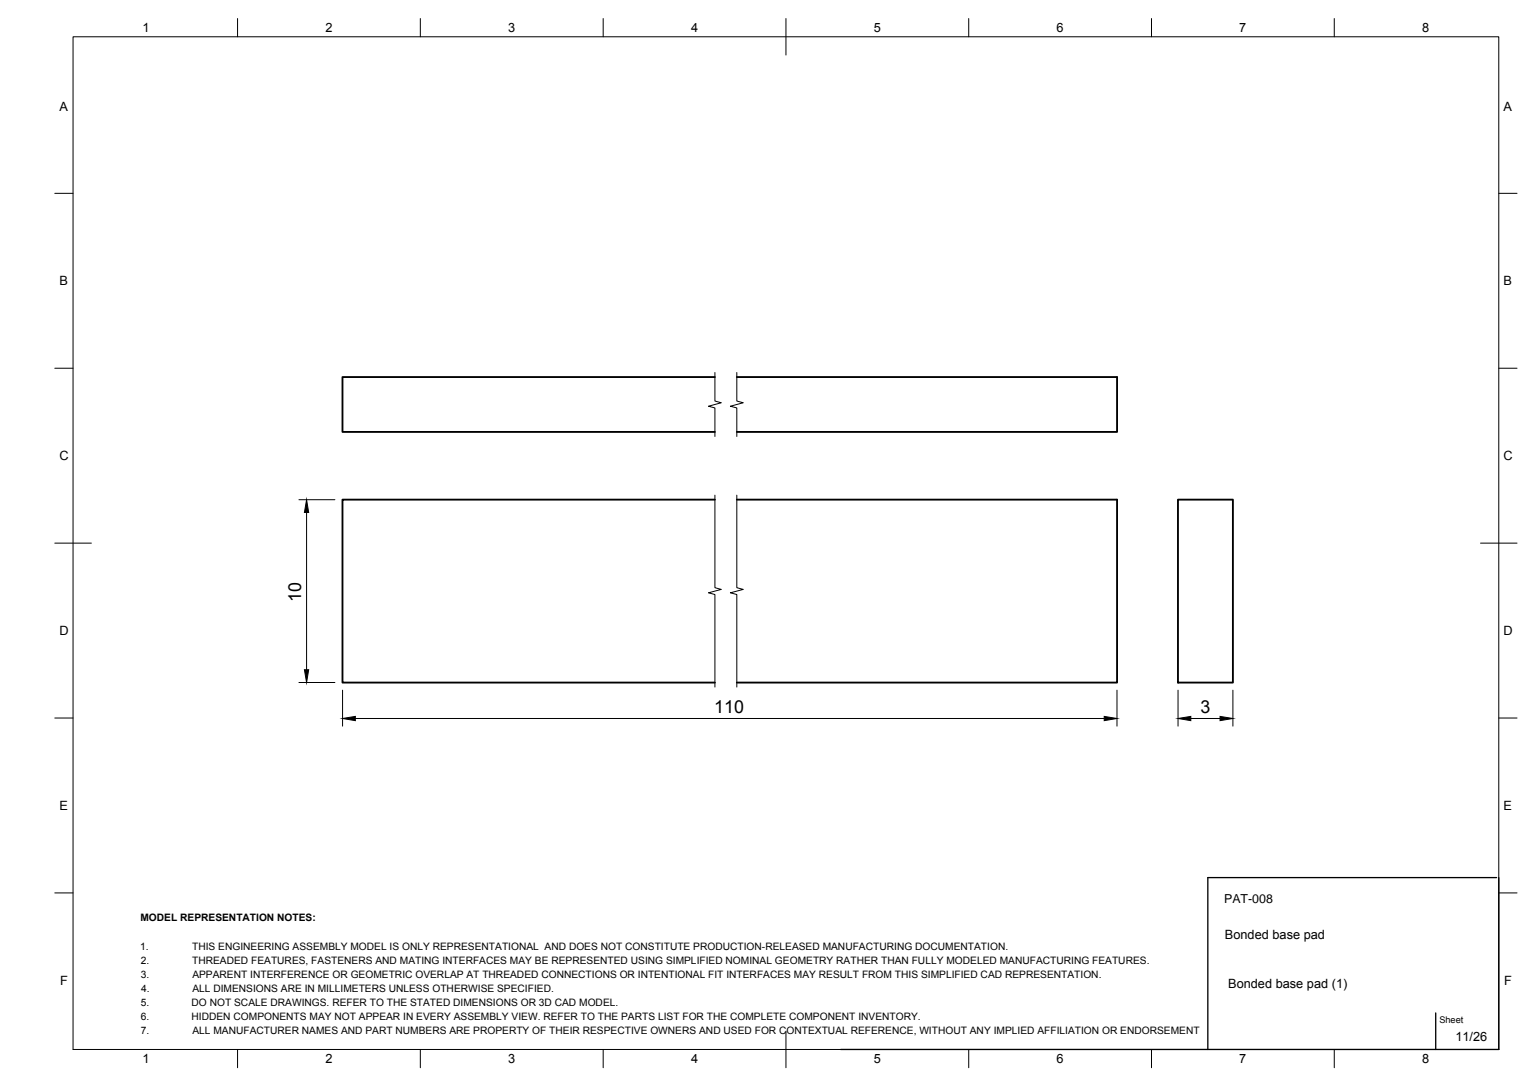
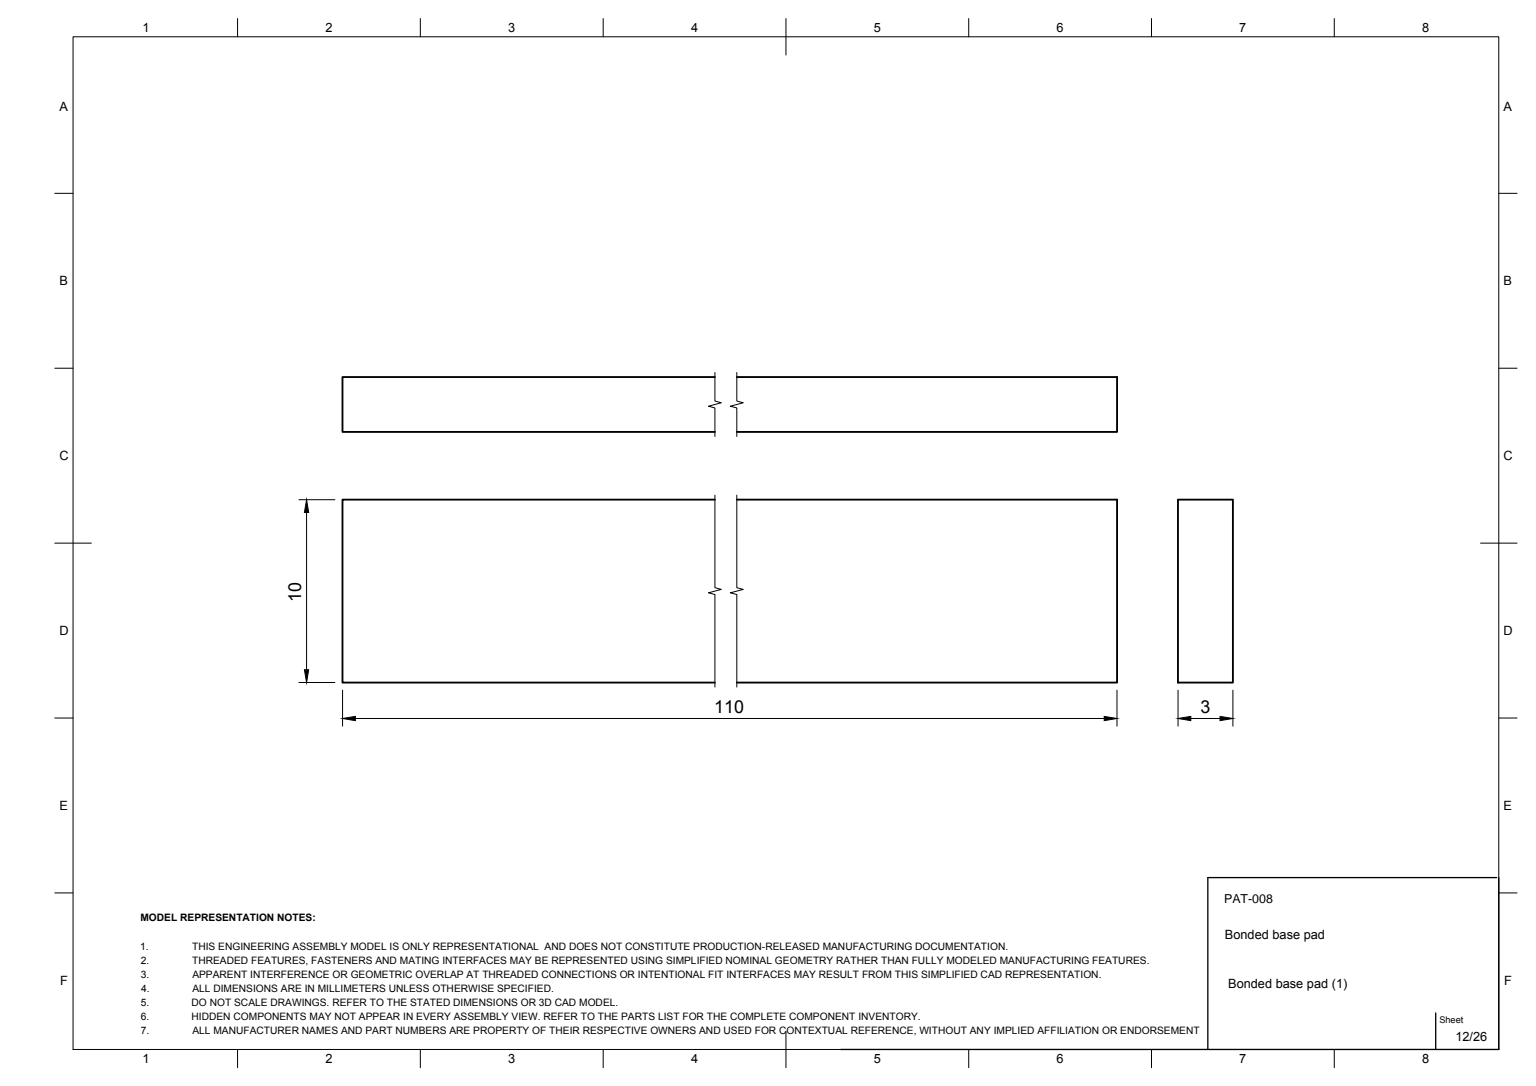
ISO-10303-21;
HEADER;
/* Generated by software containing ST-Developer
 * from STEP Tools, Inc. (www.steptools.com) 
 */

FILE_DESCRIPTION(
/* description */ ('Bearing housing with oil seal and end cap'),
/* implementation_level */ '2;1');

FILE_NAME(
/* name */ 'Bonded base pad (1).step',
/* time_stamp */ '2026-10-28T03:23:10-07:00',
/* author */ (''),
/* organization */ (''),
/* preprocessor_version */ 'ST-DEVELOPER v20.2',
/* originating_system */ 'Autodesk Translation Framework v15.17.0.0',
/* authorisation */ '');

FILE_SCHEMA (('AUTOMOTIVE_DESIGN { 1 0 10303 214 3 1 1 }'));
ENDSEC;

DATA;
#10=MECHANICAL_DESIGN_GEOMETRIC_PRESENTATION_REPRESENTATION('',(#266),#7871);
#224=SHAPE_REPRESENTATION_RELATIONSHIP('SRR','None',#7971,#245);
#245=ADVANCED_BREP_SHAPE_REPRESENTATION('',(#295),#7855);
#266=STYLED_ITEM('',(#8132),#295);
#295=MANIFOLD_SOLID_BREP('Body1',#4092);
#465=PLANE('',#4549);
#466=PLANE('',#4550);
#467=PLANE('',#4551);
#468=PLANE('',#4552);
#469=PLANE('',#4553);
#470=PLANE('',#4554);
#651=FACE_OUTER_BOUND('',#961,.T.);
#652=FACE_OUTER_BOUND('',#962,.T.);
#653=FACE_OUTER_BOUND('',#963,.T.);
#654=FACE_OUTER_BOUND('',#964,.T.);
#655=FACE_OUTER_BOUND('',#965,.T.);
#656=FACE_OUTER_BOUND('',#966,.T.);
#961=EDGE_LOOP('',(#3131,#3132,#3133,#3134));
#962=EDGE_LOOP('',(#3135,#3136,#3137,#3138));
#963=EDGE_LOOP('',(#3139,#3140,#3141,#3142));
#964=EDGE_LOOP('',(#3143,#3144,#3145,#3146));
#965=EDGE_LOOP('',(#3147,#3148,#3149,#3150));
#966=EDGE_LOOP('',(#3151,#3152,#3153,#3154));
#1249=LINE('',#6640,#1511);
#1250=LINE('',#6642,#1512);
#1251=LINE('',#6644,#1513);
#1252=LINE('',#6645,#1514);
#1253=LINE('',#6648,#1515);
#1254=LINE('',#6650,#1516);
#1255=LINE('',#6651,#1517);
#1256=LINE('',#6654,#1518);
#1257=LINE('',#6656,#1519);
#1258=LINE('',#6657,#1520);
#1259=LINE('',#6659,#1521);
#1260=LINE('',#6660,#1522);
#1511=VECTOR('',#5386,1.);
#1512=VECTOR('',#5387,1.);
#1513=VECTOR('',#5388,1.);
#1514=VECTOR('',#5389,1.);
#1515=VECTOR('',#5392,1.);
#1516=VECTOR('',#5393,1.);
#1517=VECTOR('',#5394,1.);
#1518=VECTOR('',#5397,1.);
#1519=VECTOR('',#5398,1.);
#1520=VECTOR('',#5399,1.);
#1521=VECTOR('',#5402,1.);
#1522=VECTOR('',#5403,1.);
#2019=VERTEX_POINT('',#6638);
#2020=VERTEX_POINT('',#6639);
#2021=VERTEX_POINT('',#6641);
#2022=VERTEX_POINT('',#6643);
#2023=VERTEX_POINT('',#6647);
#2024=VERTEX_POINT('',#6649);
#2025=VERTEX_POINT('',#6653);
#2026=VERTEX_POINT('',#6655);
#2429=EDGE_CURVE('',#2019,#2020,#1249,.T.);
#2430=EDGE_CURVE('',#2020,#2021,#1250,.T.);
#2431=EDGE_CURVE('',#2022,#2021,#1251,.T.);
#2432=EDGE_CURVE('',#2019,#2022,#1252,.T.);
#2433=EDGE_CURVE('',#2023,#2019,#1253,.T.);
#2434=EDGE_CURVE('',#2024,#2022,#1254,.T.);
#2435=EDGE_CURVE('',#2023,#2024,#1255,.T.);
#2436=EDGE_CURVE('',#2025,#2023,#1256,.T.);
#2437=EDGE_CURVE('',#2026,#2024,#1257,.T.);
#2438=EDGE_CURVE('',#2025,#2026,#1258,.T.);
#2439=EDGE_CURVE('',#2020,#2025,#1259,.T.);
#2440=EDGE_CURVE('',#2021,#2026,#1260,.T.);
#3131=ORIENTED_EDGE('',*,*,#2429,.T.);
#3132=ORIENTED_EDGE('',*,*,#2430,.T.);
#3133=ORIENTED_EDGE('',*,*,#2431,.F.);
#3134=ORIENTED_EDGE('',*,*,#2432,.F.);
#3135=ORIENTED_EDGE('',*,*,#2433,.T.);
#3136=ORIENTED_EDGE('',*,*,#2432,.T.);
#3137=ORIENTED_EDGE('',*,*,#2434,.F.);
#3138=ORIENTED_EDGE('',*,*,#2435,.F.);
#3139=ORIENTED_EDGE('',*,*,#2436,.T.);
#3140=ORIENTED_EDGE('',*,*,#2435,.T.);
#3141=ORIENTED_EDGE('',*,*,#2437,.F.);
#3142=ORIENTED_EDGE('',*,*,#2438,.F.);
#3143=ORIENTED_EDGE('',*,*,#2439,.T.);
#3144=ORIENTED_EDGE('',*,*,#2438,.T.);
#3145=ORIENTED_EDGE('',*,*,#2440,.F.);
#3146=ORIENTED_EDGE('',*,*,#2430,.F.);
#3147=ORIENTED_EDGE('',*,*,#2440,.T.);
#3148=ORIENTED_EDGE('',*,*,#2437,.T.);
#3149=ORIENTED_EDGE('',*,*,#2434,.T.);
#3150=ORIENTED_EDGE('',*,*,#2431,.T.);
#3151=ORIENTED_EDGE('',*,*,#2439,.F.);
#3152=ORIENTED_EDGE('',*,*,#2429,.F.);
#3153=ORIENTED_EDGE('',*,*,#2433,.F.);
#3154=ORIENTED_EDGE('',*,*,#2436,.F.);
#3933=ADVANCED_FACE('',(#651),#465,.T.);
#3934=ADVANCED_FACE('',(#652),#466,.T.);
#3935=ADVANCED_FACE('',(#653),#467,.T.);
#3936=ADVANCED_FACE('',(#654),#468,.T.);
#3937=ADVANCED_FACE('',(#655),#469,.T.);
#3938=ADVANCED_FACE('',(#656),#470,.F.);
#4092=CLOSED_SHELL('',(#3933,#3934,#3935,#3936,#3937,#3938));
#4548=AXIS2_PLACEMENT_3D('',#6636,#5382,#5383);
#4549=AXIS2_PLACEMENT_3D('',#6637,#5384,#5385);
#4550=AXIS2_PLACEMENT_3D('',#6646,#5390,#5391);
#4551=AXIS2_PLACEMENT_3D('',#6652,#5395,#5396);
#4552=AXIS2_PLACEMENT_3D('',#6658,#5400,#5401);
#4553=AXIS2_PLACEMENT_3D('',#6661,#5404,#5405);
#4554=AXIS2_PLACEMENT_3D('',#6662,#5406,#5407);
#5382=DIRECTION('axis',(0.,0.,1.));
#5383=DIRECTION('refdir',(1.,0.,0.));
#5384=DIRECTION('center_axis',(0.,1.,0.));
#5385=DIRECTION('ref_axis',(-1.,0.,0.));
#5386=DIRECTION('',(-1.,0.,0.));
#5387=DIRECTION('',(0.,0.,1.));
#5388=DIRECTION('',(-1.,0.,0.));
#5389=DIRECTION('',(0.,0.,1.));
#5390=DIRECTION('center_axis',(1.,0.,0.));
#5391=DIRECTION('ref_axis',(0.,1.,0.));
#5392=DIRECTION('',(0.,1.,0.));
#5393=DIRECTION('',(0.,1.,0.));
#5394=DIRECTION('',(0.,0.,1.));
#5395=DIRECTION('center_axis',(0.,-1.,0.));
#5396=DIRECTION('ref_axis',(1.,0.,0.));
#5397=DIRECTION('',(1.,0.,0.));
#5398=DIRECTION('',(1.,0.,0.));
#5399=DIRECTION('',(0.,0.,1.));
#5400=DIRECTION('center_axis',(-1.,0.,0.));
#5401=DIRECTION('ref_axis',(0.,-1.,0.));
#5402=DIRECTION('',(0.,-1.,0.));
#5403=DIRECTION('',(0.,-1.,0.));
#5404=DIRECTION('center_axis',(0.,0.,1.));
#5405=DIRECTION('ref_axis',(1.,0.,0.));
#5406=DIRECTION('center_axis',(0.,0.,1.));
#5407=DIRECTION('ref_axis',(1.,0.,0.));
#6636=CARTESIAN_POINT('',(0.,0.,0.));
#6637=CARTESIAN_POINT('Origin',(5.5,7.,-0.3));
#6638=CARTESIAN_POINT('',(5.5,7.,-0.3));
#6639=CARTESIAN_POINT('',(-5.5,7.,-0.3));
#6640=CARTESIAN_POINT('',(5.5,7.,-0.3));
#6641=CARTESIAN_POINT('',(-5.5,7.,0.));
#6642=CARTESIAN_POINT('',(-5.5,7.,-0.3));
#6643=CARTESIAN_POINT('',(5.5,7.,0.));
#6644=CARTESIAN_POINT('',(5.5,7.,0.));
#6645=CARTESIAN_POINT('',(5.5,7.,-0.3));
#6646=CARTESIAN_POINT('Origin',(5.5,6.,-0.3));
#6647=CARTESIAN_POINT('',(5.5,6.,-0.3));
#6648=CARTESIAN_POINT('',(5.5,6.,-0.3));
#6649=CARTESIAN_POINT('',(5.5,6.,0.));
#6650=CARTESIAN_POINT('',(5.5,6.,0.));
#6651=CARTESIAN_POINT('',(5.5,6.,-0.3));
#6652=CARTESIAN_POINT('Origin',(-5.5,6.,-0.3));
#6653=CARTESIAN_POINT('',(-5.5,6.,-0.3));
#6654=CARTESIAN_POINT('',(-5.5,6.,-0.3));
#6655=CARTESIAN_POINT('',(-5.5,6.,0.));
#6656=CARTESIAN_POINT('',(-5.5,6.,0.));
#6657=CARTESIAN_POINT('',(-5.5,6.,-0.3));
#6658=CARTESIAN_POINT('Origin',(-5.5,7.,-0.3));
#6659=CARTESIAN_POINT('',(-5.5,7.,-0.3));
#6660=CARTESIAN_POINT('',(-5.5,7.,0.));
#6661=CARTESIAN_POINT('Origin',(0.,6.5,0.));
#6662=CARTESIAN_POINT('Origin',(0.,6.5,-0.3));
#7829=UNCERTAINTY_MEASURE_WITH_UNIT(LENGTH_MEASURE(0.001),#7872,
'DISTANCE_ACCURACY_VALUE',
'Maximum model space distance between geometric entities at asserted c
onnectivities');
#7845=UNCERTAINTY_MEASURE_WITH_UNIT(LENGTH_MEASURE(0.001),#7872,
'DISTANCE_ACCURACY_VALUE',
'Maximum model space distance between geometric entities at asserted c
onnectivities');
#7855=(
GEOMETRIC_REPRESENTATION_CONTEXT(3)
GLOBAL_UNCERTAINTY_ASSIGNED_CONTEXT((#7829))
GLOBAL_UNIT_ASSIGNED_CONTEXT((#7872,#7874,#7875))
REPRESENTATION_CONTEXT('','3D')
);
#7871=(
GEOMETRIC_REPRESENTATION_CONTEXT(3)
GLOBAL_UNCERTAINTY_ASSIGNED_CONTEXT((#7845))
GLOBAL_UNIT_ASSIGNED_CONTEXT((#7872,#7874,#7875))
REPRESENTATION_CONTEXT('','3D')
);
#7872=(
LENGTH_UNIT()
NAMED_UNIT(*)
SI_UNIT(.CENTI.,.METRE.)
);
#7874=(
NAMED_UNIT(*)
PLANE_ANGLE_UNIT()
SI_UNIT($,.RADIAN.)
);
#7875=(
NAMED_UNIT(*)
SI_UNIT($,.STERADIAN.)
SOLID_ANGLE_UNIT()
);
#7885=SHAPE_DEFINITION_REPRESENTATION(#7910,#7971);
#7910=PRODUCT_DEFINITION_SHAPE('',$,#7997);
#7971=SHAPE_REPRESENTATION('',(#4548),#7855);
#7987=PRODUCT_DEFINITION_CONTEXT('part definition',#8064,'design');
#7997=PRODUCT_DEFINITION('Bonded base pad (1)','Bonded base pad (1)',#8022,
#7987);
#8022=PRODUCT_DEFINITION_FORMATION('',$,#8075);
#8064=APPLICATION_CONTEXT(
'Core Data for Automotive Mechanical Design Process');
#8065=PRODUCT_CONTEXT('part definition',#8064,'mechanical');
#8075=PRODUCT('Bonded base pad (1)','Bonded base pad (1)',
'Bonded base pad (1)',(#8065));
#8126=COLOUR_RGB('Dark Blue',0.08,0.2,0.34);
#8127=FILL_AREA_STYLE_COLOUR('',#8126);
#8128=FILL_AREA_STYLE('',(#8127));
#8129=SURFACE_STYLE_FILL_AREA(#8128);
#8130=SURFACE_SIDE_STYLE('',(#8129));
#8131=SURFACE_STYLE_USAGE(.BOTH.,#8130);
#8132=PRESENTATION_STYLE_ASSIGNMENT((#8131));
ENDSEC;
END-ISO-10303-21;
